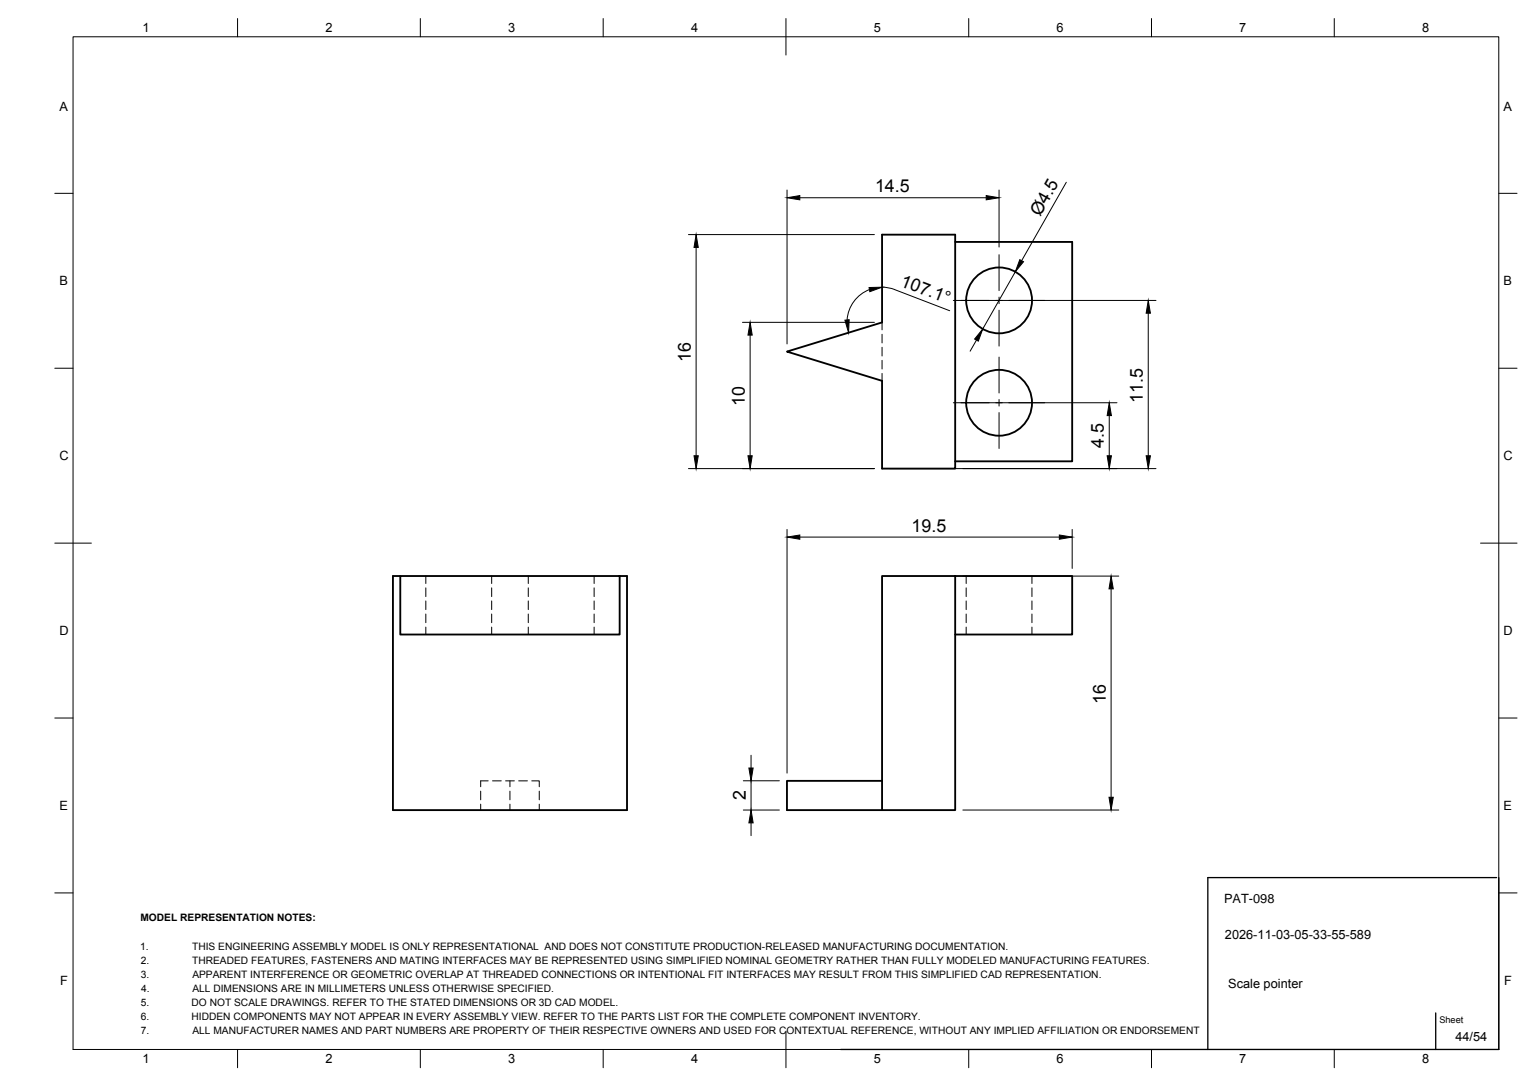
ISO-10303-21;
HEADER;
/* Generated by software containing ST-Developer
 * from STEP Tools, Inc. (www.steptools.com) 
 */

FILE_DESCRIPTION(
/* description */ ('Spring compression tester'),
/* implementation_level */ '2;1');

FILE_NAME(
/* name */ 'Scale pointer.step',
/* time_stamp */ '2026-10-28T03:24:11-07:00',
/* author */ (''),
/* organization */ (''),
/* preprocessor_version */ 'ST-DEVELOPER v20.2',
/* originating_system */ 'Autodesk Translation Framework v15.17.0.0',
/* authorisation */ '');

FILE_SCHEMA (('AUTOMOTIVE_DESIGN { 1 0 10303 214 3 1 1 }'));
ENDSEC;

DATA;
#10=MECHANICAL_DESIGN_GEOMETRIC_PRESENTATION_REPRESENTATION('',(#1163),#43521);
#1028=SHAPE_REPRESENTATION_RELATIONSHIP('SRR','None',#43843,#1088);
#1088=ADVANCED_BREP_SHAPE_REPRESENTATION('',(#1234),#43503);
#1163=STYLED_ITEM('',(#44195),#1234);
#1234=MANIFOLD_SOLID_BREP('Body1',#18604);
#1538=FACE_BOUND('',#4238,.T.);
#1539=FACE_BOUND('',#4239,.T.);
#1540=FACE_BOUND('',#4247,.T.);
#1541=FACE_BOUND('',#4248,.T.);
#2053=PLANE('',#20626);
#2054=PLANE('',#20627);
#2055=PLANE('',#20628);
#2056=PLANE('',#20629);
#2057=PLANE('',#20630);
#2058=PLANE('',#20631);
#2059=PLANE('',#20632);
#2060=PLANE('',#20633);
#2061=PLANE('',#20634);
#2062=PLANE('',#20635);
#2063=PLANE('',#20636);
#2064=PLANE('',#20637);
#2065=PLANE('',#20638);
#2893=FACE_OUTER_BOUND('',#4231,.T.);
#2894=FACE_OUTER_BOUND('',#4232,.T.);
#2895=FACE_OUTER_BOUND('',#4233,.T.);
#2896=FACE_OUTER_BOUND('',#4234,.T.);
#2897=FACE_OUTER_BOUND('',#4235,.T.);
#2898=FACE_OUTER_BOUND('',#4236,.T.);
#2899=FACE_OUTER_BOUND('',#4237,.T.);
#2900=FACE_OUTER_BOUND('',#4240,.T.);
#2901=FACE_OUTER_BOUND('',#4241,.T.);
#2902=FACE_OUTER_BOUND('',#4242,.T.);
#2903=FACE_OUTER_BOUND('',#4243,.T.);
#2904=FACE_OUTER_BOUND('',#4244,.T.);
#2905=FACE_OUTER_BOUND('',#4245,.T.);
#2906=FACE_OUTER_BOUND('',#4246,.T.);
#2907=FACE_OUTER_BOUND('',#4249,.T.);
#4231=EDGE_LOOP('',(#15501,#15502,#15503,#15504));
#4232=EDGE_LOOP('',(#15505,#15506,#15507,#15508));
#4233=EDGE_LOOP('',(#15509,#15510,#15511,#15512));
#4234=EDGE_LOOP('',(#15513,#15514,#15515,#15516));
#4235=EDGE_LOOP('',(#15517,#15518,#15519));
#4236=EDGE_LOOP('',(#15520,#15521,#15522,#15523));
#4237=EDGE_LOOP('',(#15524,#15525,#15526,#15527));
#4238=EDGE_LOOP('',(#15528));
#4239=EDGE_LOOP('',(#15529));
#4240=EDGE_LOOP('',(#15530,#15531,#15532,#15533));
#4241=EDGE_LOOP('',(#15534,#15535,#15536,#15537));
#4242=EDGE_LOOP('',(#15538,#15539,#15540,#15541,#15542,#15543,#15544,#15545));
#4243=EDGE_LOOP('',(#15546,#15547,#15548,#15549));
#4244=EDGE_LOOP('',(#15550,#15551,#15552,#15553));
#4245=EDGE_LOOP('',(#15554,#15555,#15556,#15557,#15558,#15559,#15560,#15561));
#4246=EDGE_LOOP('',(#15562,#15563,#15564,#15565,#15566,#15567,#15568,#15569));
#4247=EDGE_LOOP('',(#15570));
#4248=EDGE_LOOP('',(#15571));
#4249=EDGE_LOOP('',(#15572,#15573,#15574,#15575,#15576,#15577,#15578));
#5663=LINE('',#30619,#7095);
#5664=LINE('',#30625,#7096);
#5665=LINE('',#30630,#7097);
#5666=LINE('',#30632,#7098);
#5667=LINE('',#30634,#7099);
#5668=LINE('',#30635,#7100);
#5669=LINE('',#30638,#7101);
#5670=LINE('',#30640,#7102);
#5671=LINE('',#30641,#7103);
#5672=LINE('',#30643,#7104);
#5673=LINE('',#30647,#7105);
#5674=LINE('',#30649,#7106);
#5675=LINE('',#30651,#7107);
#5676=LINE('',#30652,#7108);
#5677=LINE('',#30655,#7109);
#5678=LINE('',#30657,#7110);
#5679=LINE('',#30658,#7111);
#5680=LINE('',#30661,#7112);
#5681=LINE('',#30663,#7113);
#5682=LINE('',#30664,#7114);
#5683=LINE('',#30666,#7115);
#5684=LINE('',#30669,#7116);
#5685=LINE('',#30671,#7117);
#5686=LINE('',#30673,#7118);
#5687=LINE('',#30675,#7119);
#5688=LINE('',#30676,#7120);
#5689=LINE('',#30679,#7121);
#5690=LINE('',#30681,#7122);
#5691=LINE('',#30682,#7123);
#5692=LINE('',#30685,#7124);
#5693=LINE('',#30687,#7125);
#5694=LINE('',#30688,#7126);
#5695=LINE('',#30690,#7127);
#5696=LINE('',#30691,#7128);
#5697=LINE('',#30692,#7129);
#7095=VECTOR('',#24929,0.225);
#7096=VECTOR('',#24936,0.225);
#7097=VECTOR('',#24941,1.);
#7098=VECTOR('',#24942,1.);
#7099=VECTOR('',#24943,1.);
#7100=VECTOR('',#24944,1.);
#7101=VECTOR('',#24947,1.);
#7102=VECTOR('',#24948,1.);
#7103=VECTOR('',#24949,1.);
#7104=VECTOR('',#24952,1.);
#7105=VECTOR('',#24955,1.);
#7106=VECTOR('',#24956,1.);
#7107=VECTOR('',#24957,1.);
#7108=VECTOR('',#24958,1.);
#7109=VECTOR('',#24961,1.);
#7110=VECTOR('',#24962,1.);
#7111=VECTOR('',#24963,1.);
#7112=VECTOR('',#24966,1.);
#7113=VECTOR('',#24967,1.);
#7114=VECTOR('',#24968,1.);
#7115=VECTOR('',#24971,1.);
#7116=VECTOR('',#24974,1.);
#7117=VECTOR('',#24975,1.);
#7118=VECTOR('',#24976,1.);
#7119=VECTOR('',#24977,1.);
#7120=VECTOR('',#24978,1.);
#7121=VECTOR('',#24981,1.);
#7122=VECTOR('',#24982,1.);
#7123=VECTOR('',#24983,1.);
#7124=VECTOR('',#24986,1.);
#7125=VECTOR('',#24987,1.);
#7126=VECTOR('',#24988,1.);
#7127=VECTOR('',#24991,1.);
#7128=VECTOR('',#24992,1.);
#7129=VECTOR('',#24993,1.);
#8021=CIRCLE('',#20621,0.225);
#8022=CIRCLE('',#20622,0.225);
#8023=CIRCLE('',#20624,0.225);
#8024=CIRCLE('',#20625,0.225);
#9242=VERTEX_POINT('',#30616);
#9243=VERTEX_POINT('',#30618);
#9244=VERTEX_POINT('',#30622);
#9245=VERTEX_POINT('',#30624);
#9246=VERTEX_POINT('',#30628);
#9247=VERTEX_POINT('',#30629);
#9248=VERTEX_POINT('',#30631);
#9249=VERTEX_POINT('',#30633);
#9250=VERTEX_POINT('',#30637);
#9251=VERTEX_POINT('',#30639);
#9252=VERTEX_POINT('',#30645);
#9253=VERTEX_POINT('',#30646);
#9254=VERTEX_POINT('',#30648);
#9255=VERTEX_POINT('',#30650);
#9256=VERTEX_POINT('',#30654);
#9257=VERTEX_POINT('',#30656);
#9258=VERTEX_POINT('',#30660);
#9259=VERTEX_POINT('',#30662);
#9260=VERTEX_POINT('',#30668);
#9261=VERTEX_POINT('',#30670);
#9262=VERTEX_POINT('',#30672);
#9263=VERTEX_POINT('',#30674);
#9264=VERTEX_POINT('',#30678);
#9265=VERTEX_POINT('',#30680);
#9266=VERTEX_POINT('',#30684);
#9267=VERTEX_POINT('',#30686);
#11415=EDGE_CURVE('',#9242,#9242,#8021,.T.);
#11416=EDGE_CURVE('',#9242,#9243,#5663,.T.);
#11417=EDGE_CURVE('',#9243,#9243,#8022,.T.);
#11418=EDGE_CURVE('',#9244,#9244,#8023,.T.);
#11419=EDGE_CURVE('',#9244,#9245,#5664,.T.);
#11420=EDGE_CURVE('',#9245,#9245,#8024,.T.);
#11421=EDGE_CURVE('',#9246,#9247,#5665,.T.);
#11422=EDGE_CURVE('',#9248,#9247,#5666,.T.);
#11423=EDGE_CURVE('',#9249,#9248,#5667,.T.);
#11424=EDGE_CURVE('',#9246,#9249,#5668,.T.);
#11425=EDGE_CURVE('',#9250,#9246,#5669,.T.);
#11426=EDGE_CURVE('',#9251,#9249,#5670,.T.);
#11427=EDGE_CURVE('',#9250,#9251,#5671,.T.);
#11428=EDGE_CURVE('',#9251,#9248,#5672,.T.);
#11429=EDGE_CURVE('',#9252,#9253,#5673,.T.);
#11430=EDGE_CURVE('',#9252,#9254,#5674,.T.);
#11431=EDGE_CURVE('',#9254,#9255,#5675,.T.);
#11432=EDGE_CURVE('',#9253,#9255,#5676,.T.);
#11433=EDGE_CURVE('',#9256,#9252,#5677,.T.);
#11434=EDGE_CURVE('',#9257,#9256,#5678,.T.);
#11435=EDGE_CURVE('',#9254,#9257,#5679,.T.);
#11436=EDGE_CURVE('',#9258,#9256,#5680,.T.);
#11437=EDGE_CURVE('',#9259,#9258,#5681,.T.);
#11438=EDGE_CURVE('',#9257,#9259,#5682,.T.);
#11439=EDGE_CURVE('',#9255,#9259,#5683,.T.);
#11440=EDGE_CURVE('',#9247,#9260,#5684,.T.);
#11441=EDGE_CURVE('',#9260,#9261,#5685,.T.);
#11442=EDGE_CURVE('',#9262,#9261,#5686,.T.);
#11443=EDGE_CURVE('',#9263,#9262,#5687,.T.);
#11444=EDGE_CURVE('',#9263,#9250,#5688,.T.);
#11445=EDGE_CURVE('',#9260,#9264,#5689,.T.);
#11446=EDGE_CURVE('',#9264,#9265,#5690,.T.);
#11447=EDGE_CURVE('',#9261,#9265,#5691,.T.);
#11448=EDGE_CURVE('',#9266,#9263,#5692,.T.);
#11449=EDGE_CURVE('',#9267,#9262,#5693,.T.);
#11450=EDGE_CURVE('',#9266,#9267,#5694,.T.);
#11451=EDGE_CURVE('',#9265,#9253,#5695,.T.);
#11452=EDGE_CURVE('',#9264,#9266,#5696,.T.);
#11453=EDGE_CURVE('',#9258,#9267,#5697,.T.);
#15501=ORIENTED_EDGE('',*,*,#11415,.F.);
#15502=ORIENTED_EDGE('',*,*,#11416,.T.);
#15503=ORIENTED_EDGE('',*,*,#11417,.F.);
#15504=ORIENTED_EDGE('',*,*,#11416,.F.);
#15505=ORIENTED_EDGE('',*,*,#11418,.F.);
#15506=ORIENTED_EDGE('',*,*,#11419,.T.);
#15507=ORIENTED_EDGE('',*,*,#11420,.F.);
#15508=ORIENTED_EDGE('',*,*,#11419,.F.);
#15509=ORIENTED_EDGE('',*,*,#11421,.T.);
#15510=ORIENTED_EDGE('',*,*,#11422,.F.);
#15511=ORIENTED_EDGE('',*,*,#11423,.F.);
#15512=ORIENTED_EDGE('',*,*,#11424,.F.);
#15513=ORIENTED_EDGE('',*,*,#11425,.T.);
#15514=ORIENTED_EDGE('',*,*,#11424,.T.);
#15515=ORIENTED_EDGE('',*,*,#11426,.F.);
#15516=ORIENTED_EDGE('',*,*,#11427,.F.);
#15517=ORIENTED_EDGE('',*,*,#11428,.F.);
#15518=ORIENTED_EDGE('',*,*,#11426,.T.);
#15519=ORIENTED_EDGE('',*,*,#11423,.T.);
#15520=ORIENTED_EDGE('',*,*,#11429,.F.);
#15521=ORIENTED_EDGE('',*,*,#11430,.T.);
#15522=ORIENTED_EDGE('',*,*,#11431,.T.);
#15523=ORIENTED_EDGE('',*,*,#11432,.F.);
#15524=ORIENTED_EDGE('',*,*,#11433,.F.);
#15525=ORIENTED_EDGE('',*,*,#11434,.F.);
#15526=ORIENTED_EDGE('',*,*,#11435,.F.);
#15527=ORIENTED_EDGE('',*,*,#11430,.F.);
#15528=ORIENTED_EDGE('',*,*,#11415,.T.);
#15529=ORIENTED_EDGE('',*,*,#11418,.T.);
#15530=ORIENTED_EDGE('',*,*,#11436,.F.);
#15531=ORIENTED_EDGE('',*,*,#11437,.F.);
#15532=ORIENTED_EDGE('',*,*,#11438,.F.);
#15533=ORIENTED_EDGE('',*,*,#11434,.T.);
#15534=ORIENTED_EDGE('',*,*,#11435,.T.);
#15535=ORIENTED_EDGE('',*,*,#11438,.T.);
#15536=ORIENTED_EDGE('',*,*,#11439,.F.);
#15537=ORIENTED_EDGE('',*,*,#11431,.F.);
#15538=ORIENTED_EDGE('',*,*,#11422,.T.);
#15539=ORIENTED_EDGE('',*,*,#11440,.T.);
#15540=ORIENTED_EDGE('',*,*,#11441,.T.);
#15541=ORIENTED_EDGE('',*,*,#11442,.F.);
#15542=ORIENTED_EDGE('',*,*,#11443,.F.);
#15543=ORIENTED_EDGE('',*,*,#11444,.T.);
#15544=ORIENTED_EDGE('',*,*,#11427,.T.);
#15545=ORIENTED_EDGE('',*,*,#11428,.T.);
#15546=ORIENTED_EDGE('',*,*,#11445,.T.);
#15547=ORIENTED_EDGE('',*,*,#11446,.T.);
#15548=ORIENTED_EDGE('',*,*,#11447,.F.);
#15549=ORIENTED_EDGE('',*,*,#11441,.F.);
#15550=ORIENTED_EDGE('',*,*,#11448,.T.);
#15551=ORIENTED_EDGE('',*,*,#11443,.T.);
#15552=ORIENTED_EDGE('',*,*,#11449,.F.);
#15553=ORIENTED_EDGE('',*,*,#11450,.F.);
#15554=ORIENTED_EDGE('',*,*,#11429,.T.);
#15555=ORIENTED_EDGE('',*,*,#11451,.F.);
#15556=ORIENTED_EDGE('',*,*,#11446,.F.);
#15557=ORIENTED_EDGE('',*,*,#11452,.T.);
#15558=ORIENTED_EDGE('',*,*,#11450,.T.);
#15559=ORIENTED_EDGE('',*,*,#11453,.F.);
#15560=ORIENTED_EDGE('',*,*,#11436,.T.);
#15561=ORIENTED_EDGE('',*,*,#11433,.T.);
#15562=ORIENTED_EDGE('',*,*,#11442,.T.);
#15563=ORIENTED_EDGE('',*,*,#11447,.T.);
#15564=ORIENTED_EDGE('',*,*,#11451,.T.);
#15565=ORIENTED_EDGE('',*,*,#11432,.T.);
#15566=ORIENTED_EDGE('',*,*,#11439,.T.);
#15567=ORIENTED_EDGE('',*,*,#11437,.T.);
#15568=ORIENTED_EDGE('',*,*,#11453,.T.);
#15569=ORIENTED_EDGE('',*,*,#11449,.T.);
#15570=ORIENTED_EDGE('',*,*,#11417,.T.);
#15571=ORIENTED_EDGE('',*,*,#11420,.T.);
#15572=ORIENTED_EDGE('',*,*,#11452,.F.);
#15573=ORIENTED_EDGE('',*,*,#11445,.F.);
#15574=ORIENTED_EDGE('',*,*,#11440,.F.);
#15575=ORIENTED_EDGE('',*,*,#11421,.F.);
#15576=ORIENTED_EDGE('',*,*,#11425,.F.);
#15577=ORIENTED_EDGE('',*,*,#11444,.F.);
#15578=ORIENTED_EDGE('',*,*,#11448,.F.);
#17304=CYLINDRICAL_SURFACE('',#20620,0.225);
#17305=CYLINDRICAL_SURFACE('',#20623,0.225);
#18217=ADVANCED_FACE('',(#2893),#17304,.F.);
#18218=ADVANCED_FACE('',(#2894),#17305,.F.);
#18219=ADVANCED_FACE('',(#2895),#2053,.T.);
#18220=ADVANCED_FACE('',(#2896),#2054,.T.);
#18221=ADVANCED_FACE('',(#2897),#2055,.T.);
#18222=ADVANCED_FACE('',(#2898),#2056,.T.);
#18223=ADVANCED_FACE('',(#2899,#1538,#1539),#2057,.F.);
#18224=ADVANCED_FACE('',(#2900),#2058,.T.);
#18225=ADVANCED_FACE('',(#2901),#2059,.T.);
#18226=ADVANCED_FACE('',(#2902),#2060,.T.);
#18227=ADVANCED_FACE('',(#2903),#2061,.T.);
#18228=ADVANCED_FACE('',(#2904),#2062,.T.);
#18229=ADVANCED_FACE('',(#2905),#2063,.T.);
#18230=ADVANCED_FACE('',(#2906,#1540,#1541),#2064,.T.);
#18231=ADVANCED_FACE('',(#2907),#2065,.F.);
#18604=CLOSED_SHELL('',(#18217,#18218,#18219,#18220,#18221,#18222,#18223,
#18224,#18225,#18226,#18227,#18228,#18229,#18230,#18231));
#20619=AXIS2_PLACEMENT_3D('',#30614,#24923,#24924);
#20620=AXIS2_PLACEMENT_3D('',#30615,#24925,#24926);
#20621=AXIS2_PLACEMENT_3D('',#30617,#24927,#24928);
#20622=AXIS2_PLACEMENT_3D('',#30620,#24930,#24931);
#20623=AXIS2_PLACEMENT_3D('',#30621,#24932,#24933);
#20624=AXIS2_PLACEMENT_3D('',#30623,#24934,#24935);
#20625=AXIS2_PLACEMENT_3D('',#30626,#24937,#24938);
#20626=AXIS2_PLACEMENT_3D('',#30627,#24939,#24940);
#20627=AXIS2_PLACEMENT_3D('',#30636,#24945,#24946);
#20628=AXIS2_PLACEMENT_3D('',#30642,#24950,#24951);
#20629=AXIS2_PLACEMENT_3D('',#30644,#24953,#24954);
#20630=AXIS2_PLACEMENT_3D('',#30653,#24959,#24960);
#20631=AXIS2_PLACEMENT_3D('',#30659,#24964,#24965);
#20632=AXIS2_PLACEMENT_3D('',#30665,#24969,#24970);
#20633=AXIS2_PLACEMENT_3D('',#30667,#24972,#24973);
#20634=AXIS2_PLACEMENT_3D('',#30677,#24979,#24980);
#20635=AXIS2_PLACEMENT_3D('',#30683,#24984,#24985);
#20636=AXIS2_PLACEMENT_3D('',#30689,#24989,#24990);
#20637=AXIS2_PLACEMENT_3D('',#30693,#24994,#24995);
#20638=AXIS2_PLACEMENT_3D('',#30694,#24996,#24997);
#24923=DIRECTION('axis',(0.,0.,1.));
#24924=DIRECTION('refdir',(1.,0.,0.));
#24925=DIRECTION('center_axis',(0.,0.,1.));
#24926=DIRECTION('ref_axis',(1.,0.,0.));
#24927=DIRECTION('center_axis',(0.,0.,1.));
#24928=DIRECTION('ref_axis',(1.,0.,0.));
#24929=DIRECTION('',(0.,0.,1.));
#24930=DIRECTION('center_axis',(0.,0.,-1.));
#24931=DIRECTION('ref_axis',(1.,0.,0.));
#24932=DIRECTION('center_axis',(0.,0.,1.));
#24933=DIRECTION('ref_axis',(1.,0.,0.));
#24934=DIRECTION('center_axis',(0.,0.,1.));
#24935=DIRECTION('ref_axis',(1.,0.,0.));
#24936=DIRECTION('',(0.,0.,1.));
#24937=DIRECTION('center_axis',(0.,0.,-1.));
#24938=DIRECTION('ref_axis',(1.,0.,0.));
#24939=DIRECTION('center_axis',(0.294085848837523,0.95577900872195,0.));
#24940=DIRECTION('ref_axis',(-0.95577900872195,0.294085848837523,0.));
#24941=DIRECTION('',(-0.95577900872195,0.294085848837523,0.));
#24942=DIRECTION('',(0.,0.,-1.));
#24943=DIRECTION('',(-0.95577900872195,0.294085848837523,0.));
#24944=DIRECTION('',(0.,0.,1.));
#24945=DIRECTION('center_axis',(0.294085848837523,-0.95577900872195,0.));
#24946=DIRECTION('ref_axis',(0.95577900872195,0.294085848837523,0.));
#24947=DIRECTION('',(0.95577900872195,0.294085848837523,0.));
#24948=DIRECTION('',(0.95577900872195,0.294085848837523,0.));
#24949=DIRECTION('',(0.,0.,1.));
#24950=DIRECTION('center_axis',(0.,0.,1.));
#24951=DIRECTION('ref_axis',(1.,0.,0.));
#24952=DIRECTION('',(0.,1.,0.));
#24953=DIRECTION('center_axis',(0.,1.,0.));
#24954=DIRECTION('ref_axis',(-1.,0.,0.));
#24955=DIRECTION('',(0.,0.,1.));
#24956=DIRECTION('',(-1.,0.,0.));
#24957=DIRECTION('',(0.,0.,1.));
#24958=DIRECTION('',(-1.,0.,0.));
#24959=DIRECTION('center_axis',(0.,0.,1.));
#24960=DIRECTION('ref_axis',(1.,0.,0.));
#24961=DIRECTION('',(0.,1.,0.));
#24962=DIRECTION('',(1.,0.,0.));
#24963=DIRECTION('',(0.,-1.,0.));
#24964=DIRECTION('center_axis',(0.,-1.,0.));
#24965=DIRECTION('ref_axis',(1.,0.,0.));
#24966=DIRECTION('',(0.,0.,-1.));
#24967=DIRECTION('',(1.,0.,0.));
#24968=DIRECTION('',(0.,0.,1.));
#24969=DIRECTION('center_axis',(-1.,0.,0.));
#24970=DIRECTION('ref_axis',(0.,-1.,0.));
#24971=DIRECTION('',(0.,-1.,0.));
#24972=DIRECTION('center_axis',(1.,0.,0.));
#24973=DIRECTION('ref_axis',(0.,1.,0.));
#24974=DIRECTION('',(0.,1.,0.));
#24975=DIRECTION('',(0.,0.,1.));
#24976=DIRECTION('',(0.,1.,0.));
#24977=DIRECTION('',(0.,0.,1.));
#24978=DIRECTION('',(0.,1.,0.));
#24979=DIRECTION('center_axis',(0.,1.,0.));
#24980=DIRECTION('ref_axis',(-1.,0.,0.));
#24981=DIRECTION('',(-1.,0.,0.));
#24982=DIRECTION('',(0.,0.,1.));
#24983=DIRECTION('',(-1.,0.,0.));
#24984=DIRECTION('center_axis',(0.,-1.,0.));
#24985=DIRECTION('ref_axis',(1.,0.,0.));
#24986=DIRECTION('',(1.,0.,0.));
#24987=DIRECTION('',(1.,0.,0.));
#24988=DIRECTION('',(0.,0.,1.));
#24989=DIRECTION('center_axis',(-1.,0.,0.));
#24990=DIRECTION('ref_axis',(0.,-1.,0.));
#24991=DIRECTION('',(0.,-1.,0.));
#24992=DIRECTION('',(0.,-1.,0.));
#24993=DIRECTION('',(0.,-1.,0.));
#24994=DIRECTION('center_axis',(0.,0.,1.));
#24995=DIRECTION('ref_axis',(1.,0.,0.));
#24996=DIRECTION('center_axis',(0.,0.,1.));
#24997=DIRECTION('ref_axis',(1.,0.,0.));
#30614=CARTESIAN_POINT('',(0.,0.,0.));
#30615=CARTESIAN_POINT('Origin',(7.2,-0.35,16.2));
#30616=CARTESIAN_POINT('',(6.975,-0.35,16.3));
#30617=CARTESIAN_POINT('Origin',(7.2,-0.35,16.3));
#30618=CARTESIAN_POINT('',(6.975,-0.35,16.7));
#30619=CARTESIAN_POINT('',(6.975,-0.35,16.2));
#30620=CARTESIAN_POINT('Origin',(7.2,-0.35,16.7));
#30621=CARTESIAN_POINT('Origin',(7.2,0.35,16.2));
#30622=CARTESIAN_POINT('',(6.975,0.35,16.3));
#30623=CARTESIAN_POINT('Origin',(7.2,0.35,16.3));
#30624=CARTESIAN_POINT('',(6.975,0.35,16.7));
#30625=CARTESIAN_POINT('',(6.975,0.35,16.2));
#30626=CARTESIAN_POINT('Origin',(7.2,0.35,16.7));
#30627=CARTESIAN_POINT('Origin',(8.65,0.,15.1));
#30628=CARTESIAN_POINT('',(8.65,0.,15.1));
#30629=CARTESIAN_POINT('',(8.,0.2,15.1));
#30630=CARTESIAN_POINT('',(8.65,0.,15.1));
#30631=CARTESIAN_POINT('',(8.,0.2,15.3));
#30632=CARTESIAN_POINT('',(8.,0.2,15.1));
#30633=CARTESIAN_POINT('',(8.65,0.,15.3));
#30634=CARTESIAN_POINT('',(8.65,0.,15.3));
#30635=CARTESIAN_POINT('',(8.65,0.,15.1));
#30636=CARTESIAN_POINT('Origin',(8.,-0.2,15.1));
#30637=CARTESIAN_POINT('',(8.,-0.2,15.1));
#30638=CARTESIAN_POINT('',(8.,-0.2,15.1));
#30639=CARTESIAN_POINT('',(8.,-0.2,15.3));
#30640=CARTESIAN_POINT('',(8.,-0.2,15.3));
#30641=CARTESIAN_POINT('',(8.,-0.2,15.1));
#30642=CARTESIAN_POINT('Origin',(8.325,0.,15.3));
#30643=CARTESIAN_POINT('',(8.,-0.4,15.3));
#30644=CARTESIAN_POINT('Origin',(8.,0.75,16.3));
#30645=CARTESIAN_POINT('',(7.5,0.75,16.3));
#30646=CARTESIAN_POINT('',(7.5,0.75,16.7));
#30647=CARTESIAN_POINT('',(7.5,0.75,15.7));
#30648=CARTESIAN_POINT('',(6.7,0.75,16.3));
#30649=CARTESIAN_POINT('',(8.,0.75,16.3));
#30650=CARTESIAN_POINT('',(6.7,0.75,16.7));
#30651=CARTESIAN_POINT('',(6.7,0.75,16.3));
#30652=CARTESIAN_POINT('',(8.,0.75,16.7));
#30653=CARTESIAN_POINT('Origin',(7.35,0.,16.3));
#30654=CARTESIAN_POINT('',(7.5,-0.75,16.3));
#30655=CARTESIAN_POINT('',(7.5,0.4,16.3));
#30656=CARTESIAN_POINT('',(6.7,-0.75,16.3));
#30657=CARTESIAN_POINT('',(6.7,-0.75,16.3));
#30658=CARTESIAN_POINT('',(6.7,0.75,16.3));
#30659=CARTESIAN_POINT('Origin',(6.7,-0.75,16.3));
#30660=CARTESIAN_POINT('',(7.5,-0.75,16.7));
#30661=CARTESIAN_POINT('',(7.5,-0.75,15.7));
#30662=CARTESIAN_POINT('',(6.7,-0.75,16.7));
#30663=CARTESIAN_POINT('',(6.7,-0.75,16.7));
#30664=CARTESIAN_POINT('',(6.7,-0.75,16.3));
#30665=CARTESIAN_POINT('Origin',(6.7,0.75,16.3));
#30666=CARTESIAN_POINT('',(6.7,0.75,16.7));
#30667=CARTESIAN_POINT('Origin',(8.,-0.8,15.1));
#30668=CARTESIAN_POINT('',(8.,0.8,15.1));
#30669=CARTESIAN_POINT('',(8.,-0.8,15.1));
#30670=CARTESIAN_POINT('',(8.,0.8,16.7));
#30671=CARTESIAN_POINT('',(8.,0.8,15.1));
#30672=CARTESIAN_POINT('',(8.,-0.8,16.7));
#30673=CARTESIAN_POINT('',(8.,-0.8,16.7));
#30674=CARTESIAN_POINT('',(8.,-0.8,15.1));
#30675=CARTESIAN_POINT('',(8.,-0.8,15.1));
#30676=CARTESIAN_POINT('',(8.,-0.8,15.1));
#30677=CARTESIAN_POINT('Origin',(8.,0.8,15.1));
#30678=CARTESIAN_POINT('',(7.5,0.8,15.1));
#30679=CARTESIAN_POINT('',(8.,0.8,15.1));
#30680=CARTESIAN_POINT('',(7.5,0.8,16.7));
#30681=CARTESIAN_POINT('',(7.5,0.8,15.1));
#30682=CARTESIAN_POINT('',(8.,0.8,16.7));
#30683=CARTESIAN_POINT('Origin',(7.5,-0.8,15.1));
#30684=CARTESIAN_POINT('',(7.5,-0.8,15.1));
#30685=CARTESIAN_POINT('',(7.5,-0.8,15.1));
#30686=CARTESIAN_POINT('',(7.5,-0.8,16.7));
#30687=CARTESIAN_POINT('',(7.5,-0.8,16.7));
#30688=CARTESIAN_POINT('',(7.5,-0.8,15.1));
#30689=CARTESIAN_POINT('Origin',(7.5,0.8,15.1));
#30690=CARTESIAN_POINT('',(7.5,0.8,16.7));
#30691=CARTESIAN_POINT('',(7.5,0.8,15.1));
#30692=CARTESIAN_POINT('',(7.5,0.8,16.7));
#30693=CARTESIAN_POINT('Origin',(7.75,0.,16.7));
#30694=CARTESIAN_POINT('Origin',(7.75,0.,15.1));
#43435=UNCERTAINTY_MEASURE_WITH_UNIT(LENGTH_MEASURE(0.001),#43522,
'DISTANCE_ACCURACY_VALUE',
'Maximum model space distance between geometric entities at asserted c
onnectivities');
#43453=UNCERTAINTY_MEASURE_WITH_UNIT(LENGTH_MEASURE(0.001),#43522,
'DISTANCE_ACCURACY_VALUE',
'Maximum model space distance between geometric entities at asserted c
onnectivities');
#43503=(
GEOMETRIC_REPRESENTATION_CONTEXT(3)
GLOBAL_UNCERTAINTY_ASSIGNED_CONTEXT((#43435))
GLOBAL_UNIT_ASSIGNED_CONTEXT((#43522,#43524,#43525))
REPRESENTATION_CONTEXT('','3D')
);
#43521=(
GEOMETRIC_REPRESENTATION_CONTEXT(3)
GLOBAL_UNCERTAINTY_ASSIGNED_CONTEXT((#43453))
GLOBAL_UNIT_ASSIGNED_CONTEXT((#43522,#43524,#43525))
REPRESENTATION_CONTEXT('','3D')
);
#43522=(
LENGTH_UNIT()
NAMED_UNIT(*)
SI_UNIT(.CENTI.,.METRE.)
);
#43524=(
NAMED_UNIT(*)
PLANE_ANGLE_UNIT()
SI_UNIT($,.RADIAN.)
);
#43525=(
NAMED_UNIT(*)
SI_UNIT($,.STERADIAN.)
SOLID_ANGLE_UNIT()
);
#43575=SHAPE_DEFINITION_REPRESENTATION(#43652,#43843);
#43652=PRODUCT_DEFINITION_SHAPE('',$,#43911);
#43843=SHAPE_REPRESENTATION('',(#20619),#43503);
#43861=PRODUCT_DEFINITION_CONTEXT('part definition',#44064,'design');
#43911=PRODUCT_DEFINITION('Scale pointer','Scale pointer',#43978,#43861);
#43978=PRODUCT_DEFINITION_FORMATION('',$,#44115);
#44064=APPLICATION_CONTEXT(
'Core Data for Automotive Mechanical Design Process');
#44065=PRODUCT_CONTEXT('part definition',#44064,'mechanical');
#44115=PRODUCT('Scale pointer','Scale pointer','Scale pointer',(#44065));
#44189=COLOUR_RGB('Sky Blue',0.24,0.69,0.87);
#44190=FILL_AREA_STYLE_COLOUR('',#44189);
#44191=FILL_AREA_STYLE('',(#44190));
#44192=SURFACE_STYLE_FILL_AREA(#44191);
#44193=SURFACE_SIDE_STYLE('',(#44192));
#44194=SURFACE_STYLE_USAGE(.BOTH.,#44193);
#44195=PRESENTATION_STYLE_ASSIGNMENT((#44194));
ENDSEC;
END-ISO-10303-21;
